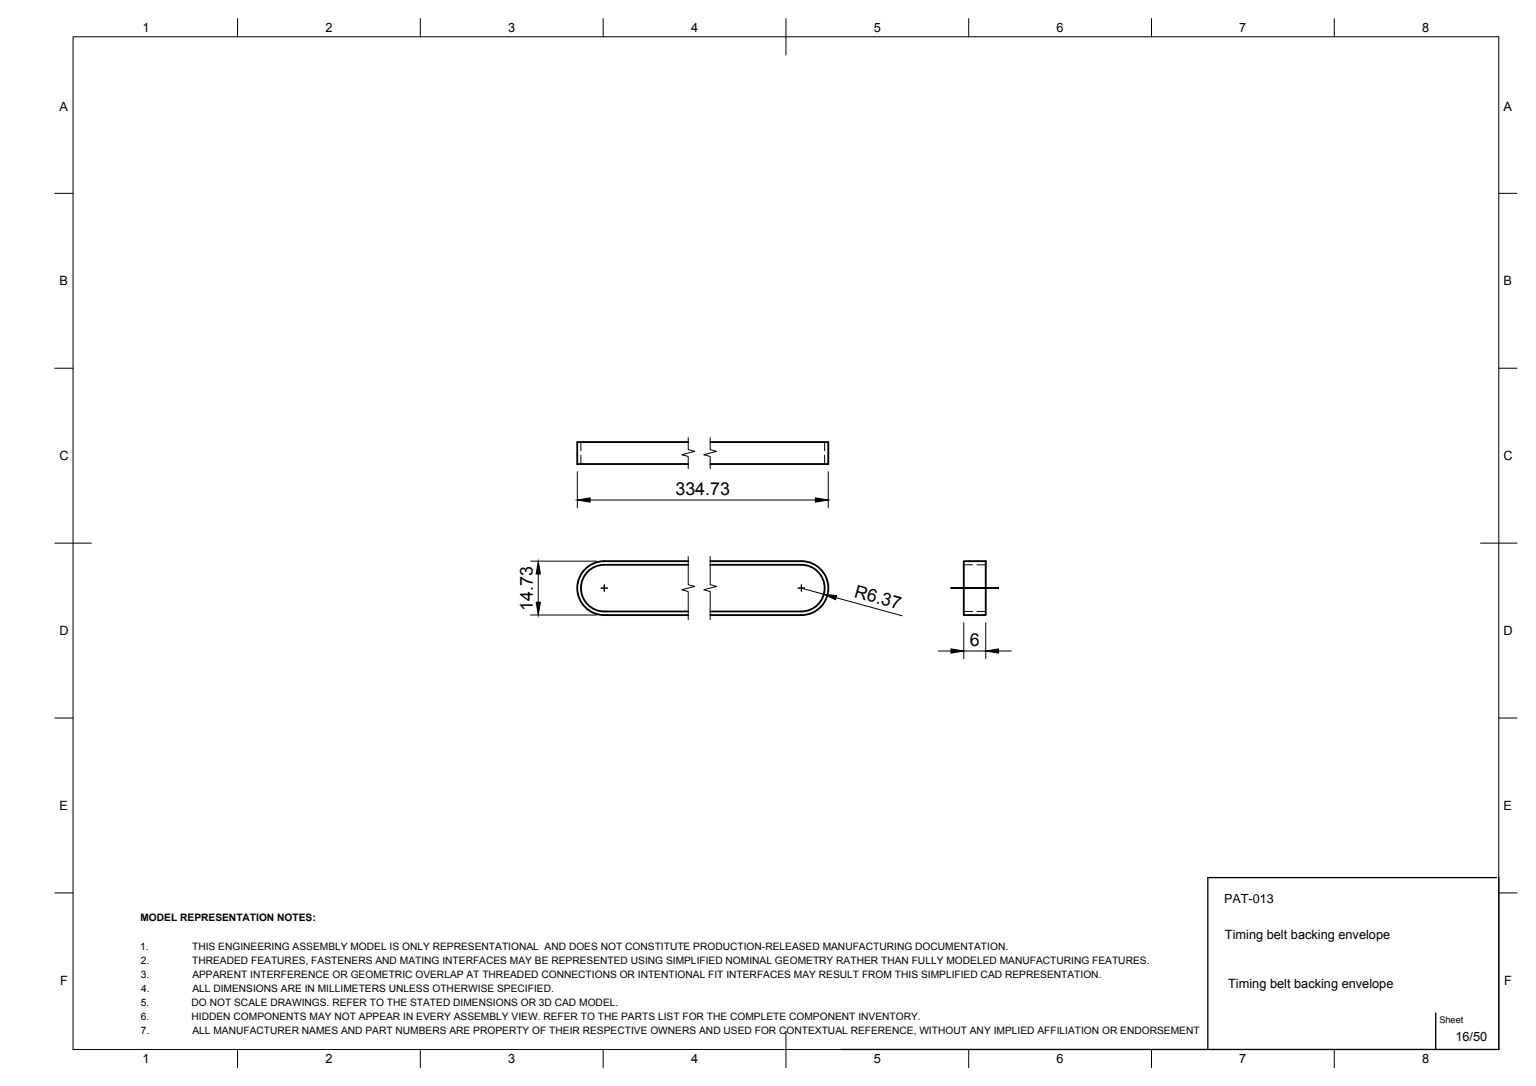
ISO-10303-21;
HEADER;
/* Generated by software containing ST-Developer
 * from STEP Tools, Inc. (www.steptools.com) 
 */

FILE_DESCRIPTION(
/* description */ ('Belt-driven linear axis on 2020 extrusion'),
/* implementation_level */ '2;1');

FILE_NAME(
/* name */ 'Timing belt backing envelope.step',
/* time_stamp */ '2026-10-28T03:26:09-07:00',
/* author */ (''),
/* organization */ (''),
/* preprocessor_version */ 'ST-DEVELOPER v20.2',
/* originating_system */ 'Autodesk Translation Framework v15.17.0.0',
/* authorisation */ '');

FILE_SCHEMA (('AUTOMOTIVE_DESIGN { 1 0 10303 214 3 1 1 }'));
ENDSEC;

DATA;
#10=MECHANICAL_DESIGN_GEOMETRIC_PRESENTATION_REPRESENTATION('',(#623),#20096);
#529=SHAPE_REPRESENTATION_RELATIONSHIP('SRR','None',#20325,#575);
#575=ADVANCED_BREP_SHAPE_REPRESENTATION('',(#679),#20056);
#623=STYLED_ITEM('',(#20657),#679);
#679=MANIFOLD_SOLID_BREP('Body1',#10936);
#794=FACE_BOUND('',#2115,.T.);
#795=FACE_BOUND('',#2123,.T.);
#971=PLANE('',#11832);
#972=PLANE('',#11833);
#973=PLANE('',#11834);
#974=PLANE('',#11845);
#975=PLANE('',#11846);
#976=PLANE('',#11849);
#1414=FACE_OUTER_BOUND('',#2112,.T.);
#1415=FACE_OUTER_BOUND('',#2113,.T.);
#1416=FACE_OUTER_BOUND('',#2114,.T.);
#1417=FACE_OUTER_BOUND('',#2116,.T.);
#1418=FACE_OUTER_BOUND('',#2117,.T.);
#1419=FACE_OUTER_BOUND('',#2118,.T.);
#1420=FACE_OUTER_BOUND('',#2119,.T.);
#1421=FACE_OUTER_BOUND('',#2120,.T.);
#1422=FACE_OUTER_BOUND('',#2121,.T.);
#1423=FACE_OUTER_BOUND('',#2122,.T.);
#2112=EDGE_LOOP('',(#7961,#7962,#7963,#7964));
#2113=EDGE_LOOP('',(#7965,#7966,#7967,#7968));
#2114=EDGE_LOOP('',(#7969,#7970,#7971,#7972));
#2115=EDGE_LOOP('',(#7973,#7974,#7975,#7976));
#2116=EDGE_LOOP('',(#7977,#7978,#7979,#7980));
#2117=EDGE_LOOP('',(#7981,#7982,#7983,#7984));
#2118=EDGE_LOOP('',(#7985,#7986,#7987,#7988));
#2119=EDGE_LOOP('',(#7989,#7990,#7991,#7992));
#2120=EDGE_LOOP('',(#7993,#7994,#7995,#7996));
#2121=EDGE_LOOP('',(#7997,#7998,#7999,#8000));
#2122=EDGE_LOOP('',(#8001,#8002,#8003,#8004));
#2123=EDGE_LOOP('',(#8005,#8006,#8007,#8008));
#2855=LINE('',#17003,#3712);
#2856=LINE('',#17005,#3713);
#2857=LINE('',#17007,#3714);
#2858=LINE('',#17008,#3715);
#2859=LINE('',#17012,#3716);
#2860=LINE('',#17014,#3717);
#2861=LINE('',#17016,#3718);
#2862=LINE('',#17017,#3719);
#2863=LINE('',#17021,#3720);
#2864=LINE('',#17025,#3721);
#2865=LINE('',#17035,#3722);
#2866=LINE('',#17038,#3723);
#2867=LINE('',#17041,#3724);
#2868=LINE('',#17042,#3725);
#2869=LINE('',#17045,#3726);
#2870=LINE('',#17046,#3727);
#3712=VECTOR('',#13661,1.);
#3713=VECTOR('',#13662,1.);
#3714=VECTOR('',#13663,1.);
#3715=VECTOR('',#13664,1.);
#3716=VECTOR('',#13667,1.);
#3717=VECTOR('',#13668,1.);
#3718=VECTOR('',#13669,1.);
#3719=VECTOR('',#13670,1.);
#3720=VECTOR('',#13673,1.);
#3721=VECTOR('',#13676,1.);
#3722=VECTOR('',#13693,1.);
#3723=VECTOR('',#13696,1.);
#3724=VECTOR('',#13699,1.);
#3725=VECTOR('',#13700,1.);
#3726=VECTOR('',#13703,1.);
#3727=VECTOR('',#13704,1.);
#4543=CIRCLE('',#11835,0.736619772367581);
#4544=CIRCLE('',#11836,0.736619772367582);
#4545=CIRCLE('',#11837,0.636619772367581);
#4546=CIRCLE('',#11838,0.636619772367581);
#4547=CIRCLE('',#11840,0.636619772367581);
#4548=CIRCLE('',#11842,0.636619772367581);
#4549=CIRCLE('',#11844,0.736619772367582);
#4550=CIRCLE('',#11848,0.736619772367581);
#5128=VERTEX_POINT('',#17001);
#5129=VERTEX_POINT('',#17002);
#5130=VERTEX_POINT('',#17004);
#5131=VERTEX_POINT('',#17006);
#5132=VERTEX_POINT('',#17010);
#5133=VERTEX_POINT('',#17011);
#5134=VERTEX_POINT('',#17013);
#5135=VERTEX_POINT('',#17015);
#5136=VERTEX_POINT('',#17019);
#5137=VERTEX_POINT('',#17020);
#5138=VERTEX_POINT('',#17022);
#5139=VERTEX_POINT('',#17024);
#5140=VERTEX_POINT('',#17034);
#5141=VERTEX_POINT('',#17036);
#5142=VERTEX_POINT('',#17040);
#5143=VERTEX_POINT('',#17044);
#6195=EDGE_CURVE('',#5128,#5129,#2855,.T.);
#6196=EDGE_CURVE('',#5130,#5128,#2856,.T.);
#6197=EDGE_CURVE('',#5131,#5130,#2857,.T.);
#6198=EDGE_CURVE('',#5131,#5129,#2858,.T.);
#6199=EDGE_CURVE('',#5132,#5133,#2859,.T.);
#6200=EDGE_CURVE('',#5134,#5132,#2860,.T.);
#6201=EDGE_CURVE('',#5135,#5134,#2861,.T.);
#6202=EDGE_CURVE('',#5133,#5135,#2862,.T.);
#6203=EDGE_CURVE('',#5136,#5137,#2863,.T.);
#6204=EDGE_CURVE('',#5138,#5136,#4543,.T.);
#6205=EDGE_CURVE('',#5139,#5138,#2864,.T.);
#6206=EDGE_CURVE('',#5137,#5139,#4544,.T.);
#6207=EDGE_CURVE('',#5129,#5132,#4545,.T.);
#6208=EDGE_CURVE('',#5133,#5128,#4546,.T.);
#6209=EDGE_CURVE('',#5134,#5131,#4547,.T.);
#6210=EDGE_CURVE('',#5130,#5135,#4548,.T.);
#6211=EDGE_CURVE('',#5139,#5140,#2865,.T.);
#6212=EDGE_CURVE('',#5141,#5140,#4549,.T.);
#6213=EDGE_CURVE('',#5137,#5141,#2866,.T.);
#6214=EDGE_CURVE('',#5138,#5142,#2867,.T.);
#6215=EDGE_CURVE('',#5140,#5142,#2868,.T.);
#6216=EDGE_CURVE('',#5143,#5141,#2869,.T.);
#6217=EDGE_CURVE('',#5136,#5143,#2870,.T.);
#6218=EDGE_CURVE('',#5142,#5143,#4550,.T.);
#7961=ORIENTED_EDGE('',*,*,#6195,.F.);
#7962=ORIENTED_EDGE('',*,*,#6196,.F.);
#7963=ORIENTED_EDGE('',*,*,#6197,.F.);
#7964=ORIENTED_EDGE('',*,*,#6198,.T.);
#7965=ORIENTED_EDGE('',*,*,#6199,.F.);
#7966=ORIENTED_EDGE('',*,*,#6200,.F.);
#7967=ORIENTED_EDGE('',*,*,#6201,.F.);
#7968=ORIENTED_EDGE('',*,*,#6202,.F.);
#7969=ORIENTED_EDGE('',*,*,#6203,.F.);
#7970=ORIENTED_EDGE('',*,*,#6204,.F.);
#7971=ORIENTED_EDGE('',*,*,#6205,.F.);
#7972=ORIENTED_EDGE('',*,*,#6206,.F.);
#7973=ORIENTED_EDGE('',*,*,#6195,.T.);
#7974=ORIENTED_EDGE('',*,*,#6207,.T.);
#7975=ORIENTED_EDGE('',*,*,#6199,.T.);
#7976=ORIENTED_EDGE('',*,*,#6208,.T.);
#7977=ORIENTED_EDGE('',*,*,#6198,.F.);
#7978=ORIENTED_EDGE('',*,*,#6209,.F.);
#7979=ORIENTED_EDGE('',*,*,#6200,.T.);
#7980=ORIENTED_EDGE('',*,*,#6207,.F.);
#7981=ORIENTED_EDGE('',*,*,#6196,.T.);
#7982=ORIENTED_EDGE('',*,*,#6208,.F.);
#7983=ORIENTED_EDGE('',*,*,#6202,.T.);
#7984=ORIENTED_EDGE('',*,*,#6210,.F.);
#7985=ORIENTED_EDGE('',*,*,#6211,.T.);
#7986=ORIENTED_EDGE('',*,*,#6212,.F.);
#7987=ORIENTED_EDGE('',*,*,#6213,.F.);
#7988=ORIENTED_EDGE('',*,*,#6206,.T.);
#7989=ORIENTED_EDGE('',*,*,#6205,.T.);
#7990=ORIENTED_EDGE('',*,*,#6214,.T.);
#7991=ORIENTED_EDGE('',*,*,#6215,.F.);
#7992=ORIENTED_EDGE('',*,*,#6211,.F.);
#7993=ORIENTED_EDGE('',*,*,#6203,.T.);
#7994=ORIENTED_EDGE('',*,*,#6213,.T.);
#7995=ORIENTED_EDGE('',*,*,#6216,.F.);
#7996=ORIENTED_EDGE('',*,*,#6217,.F.);
#7997=ORIENTED_EDGE('',*,*,#6214,.F.);
#7998=ORIENTED_EDGE('',*,*,#6204,.T.);
#7999=ORIENTED_EDGE('',*,*,#6217,.T.);
#8000=ORIENTED_EDGE('',*,*,#6218,.F.);
#8001=ORIENTED_EDGE('',*,*,#6215,.T.);
#8002=ORIENTED_EDGE('',*,*,#6218,.T.);
#8003=ORIENTED_EDGE('',*,*,#6216,.T.);
#8004=ORIENTED_EDGE('',*,*,#6212,.T.);
#8005=ORIENTED_EDGE('',*,*,#6197,.T.);
#8006=ORIENTED_EDGE('',*,*,#6210,.T.);
#8007=ORIENTED_EDGE('',*,*,#6201,.T.);
#8008=ORIENTED_EDGE('',*,*,#6209,.T.);
#10159=CYLINDRICAL_SURFACE('',#11839,0.636619772367581);
#10160=CYLINDRICAL_SURFACE('',#11841,0.636619772367581);
#10161=CYLINDRICAL_SURFACE('',#11843,0.736619772367582);
#10162=CYLINDRICAL_SURFACE('',#11847,0.736619772367581);
#10465=ADVANCED_FACE('',(#1414),#971,.F.);
#10466=ADVANCED_FACE('',(#1415),#972,.F.);
#10467=ADVANCED_FACE('',(#1416,#794),#973,.F.);
#10468=ADVANCED_FACE('',(#1417),#10159,.F.);
#10469=ADVANCED_FACE('',(#1418),#10160,.F.);
#10470=ADVANCED_FACE('',(#1419),#10161,.T.);
#10471=ADVANCED_FACE('',(#1420),#974,.T.);
#10472=ADVANCED_FACE('',(#1421),#975,.T.);
#10473=ADVANCED_FACE('',(#1422),#10162,.T.);
#10474=ADVANCED_FACE('',(#1423,#795),#976,.T.);
#10936=CLOSED_SHELL('',(#10465,#10466,#10467,#10468,#10469,#10470,#10471,
#10472,#10473,#10474));
#11831=AXIS2_PLACEMENT_3D('',#16999,#13657,#13658);
#11832=AXIS2_PLACEMENT_3D('',#17000,#13659,#13660);
#11833=AXIS2_PLACEMENT_3D('',#17009,#13665,#13666);
#11834=AXIS2_PLACEMENT_3D('',#17018,#13671,#13672);
#11835=AXIS2_PLACEMENT_3D('',#17023,#13674,#13675);
#11836=AXIS2_PLACEMENT_3D('',#17026,#13677,#13678);
#11837=AXIS2_PLACEMENT_3D('',#17027,#13679,#13680);
#11838=AXIS2_PLACEMENT_3D('',#17028,#13681,#13682);
#11839=AXIS2_PLACEMENT_3D('',#17029,#13683,#13684);
#11840=AXIS2_PLACEMENT_3D('',#17030,#13685,#13686);
#11841=AXIS2_PLACEMENT_3D('',#17031,#13687,#13688);
#11842=AXIS2_PLACEMENT_3D('',#17032,#13689,#13690);
#11843=AXIS2_PLACEMENT_3D('',#17033,#13691,#13692);
#11844=AXIS2_PLACEMENT_3D('',#17037,#13694,#13695);
#11845=AXIS2_PLACEMENT_3D('',#17039,#13697,#13698);
#11846=AXIS2_PLACEMENT_3D('',#17043,#13701,#13702);
#11847=AXIS2_PLACEMENT_3D('',#17047,#13705,#13706);
#11848=AXIS2_PLACEMENT_3D('',#17048,#13707,#13708);
#11849=AXIS2_PLACEMENT_3D('',#17049,#13709,#13710);
#13657=DIRECTION('axis',(0.,0.,1.));
#13658=DIRECTION('refdir',(1.,0.,0.));
#13659=DIRECTION('center_axis',(0.,0.,-1.));
#13660=DIRECTION('ref_axis',(-1.,0.,0.));
#13661=DIRECTION('',(-1.,0.,0.));
#13662=DIRECTION('',(0.,-1.,0.));
#13663=DIRECTION('',(1.,0.,0.));
#13664=DIRECTION('',(0.,-1.,0.));
#13665=DIRECTION('center_axis',(0.,0.,1.));
#13666=DIRECTION('ref_axis',(1.,0.,0.));
#13667=DIRECTION('',(1.,0.,0.));
#13668=DIRECTION('',(0.,-1.,0.));
#13669=DIRECTION('',(-1.,0.,0.));
#13670=DIRECTION('',(0.,1.,0.));
#13671=DIRECTION('center_axis',(0.,1.,0.));
#13672=DIRECTION('ref_axis',(1.,0.,0.));
#13673=DIRECTION('',(1.,0.,0.));
#13674=DIRECTION('center_axis',(0.,1.,0.));
#13675=DIRECTION('ref_axis',(1.,0.,0.));
#13676=DIRECTION('',(-1.,0.,0.));
#13677=DIRECTION('center_axis',(0.,1.,0.));
#13678=DIRECTION('ref_axis',(1.,0.,0.));
#13679=DIRECTION('center_axis',(0.,1.,0.));
#13680=DIRECTION('ref_axis',(1.,0.,0.));
#13681=DIRECTION('center_axis',(0.,1.,0.));
#13682=DIRECTION('ref_axis',(1.,0.,0.));
#13683=DIRECTION('center_axis',(0.,1.,0.));
#13684=DIRECTION('ref_axis',(-1.,0.,-1.22464679914735E-16));
#13685=DIRECTION('center_axis',(0.,-1.,0.));
#13686=DIRECTION('ref_axis',(1.,0.,0.));
#13687=DIRECTION('center_axis',(0.,1.,0.));
#13688=DIRECTION('ref_axis',(1.,0.,0.));
#13689=DIRECTION('center_axis',(0.,-1.,0.));
#13690=DIRECTION('ref_axis',(1.,0.,0.));
#13691=DIRECTION('center_axis',(0.,1.,0.));
#13692=DIRECTION('ref_axis',(1.,0.,0.));
#13693=DIRECTION('',(0.,1.,0.));
#13694=DIRECTION('center_axis',(0.,1.,0.));
#13695=DIRECTION('ref_axis',(1.,0.,0.));
#13696=DIRECTION('',(0.,1.,0.));
#13697=DIRECTION('center_axis',(0.,0.,-1.));
#13698=DIRECTION('ref_axis',(-1.,0.,0.));
#13699=DIRECTION('',(0.,1.,0.));
#13700=DIRECTION('',(-1.,0.,0.));
#13701=DIRECTION('center_axis',(0.,0.,1.));
#13702=DIRECTION('ref_axis',(1.,0.,0.));
#13703=DIRECTION('',(1.,0.,0.));
#13704=DIRECTION('',(0.,1.,0.));
#13705=DIRECTION('center_axis',(0.,1.,0.));
#13706=DIRECTION('ref_axis',(-1.,0.,-1.22464679914735E-16));
#13707=DIRECTION('center_axis',(0.,1.,0.));
#13708=DIRECTION('ref_axis',(1.,0.,0.));
#13709=DIRECTION('center_axis',(0.,1.,0.));
#13710=DIRECTION('ref_axis',(1.,0.,0.));
#16999=CARTESIAN_POINT('',(0.,0.,0.));
#17000=CARTESIAN_POINT('Origin',(32.,-3.5,6.36338022763242));
#17001=CARTESIAN_POINT('',(32.,-3.425,6.36338022763242));
#17002=CARTESIAN_POINT('',(0.,-3.425,6.36338022763242));
#17003=CARTESIAN_POINT('',(16.,-3.425,6.36338022763242));
#17004=CARTESIAN_POINT('',(32.,-2.825,6.36338022763242));
#17005=CARTESIAN_POINT('',(32.,-3.5,6.36338022763242));
#17006=CARTESIAN_POINT('',(0.,-2.825,6.36338022763242));
#17007=CARTESIAN_POINT('',(16.,-2.825,6.36338022763242));
#17008=CARTESIAN_POINT('',(0.,-3.5,6.36338022763242));
#17009=CARTESIAN_POINT('Origin',(0.,-3.5,7.63661977236758));
#17010=CARTESIAN_POINT('',(0.,-3.425,7.63661977236758));
#17011=CARTESIAN_POINT('',(32.,-3.425,7.63661977236758));
#17012=CARTESIAN_POINT('',(0.,-3.425,7.63661977236758));
#17013=CARTESIAN_POINT('',(0.,-2.825,7.63661977236758));
#17014=CARTESIAN_POINT('',(0.,-3.5,7.63661977236758));
#17015=CARTESIAN_POINT('',(32.,-2.825,7.63661977236758));
#17016=CARTESIAN_POINT('',(0.,-2.825,7.63661977236758));
#17017=CARTESIAN_POINT('',(32.,-3.5,7.63661977236758));
#17018=CARTESIAN_POINT('Origin',(0.,-3.425,7.));
#17019=CARTESIAN_POINT('',(0.,-3.425,7.73661977236758));
#17020=CARTESIAN_POINT('',(32.,-3.425,7.73661977236758));
#17021=CARTESIAN_POINT('',(0.,-3.425,7.73661977236758));
#17022=CARTESIAN_POINT('',(0.,-3.425,6.26338022763242));
#17023=CARTESIAN_POINT('Origin',(0.,-3.425,7.));
#17024=CARTESIAN_POINT('',(32.,-3.425,6.26338022763242));
#17025=CARTESIAN_POINT('',(32.,-3.425,6.26338022763242));
#17026=CARTESIAN_POINT('Origin',(32.,-3.425,7.));
#17027=CARTESIAN_POINT('Origin',(0.,-3.425,7.));
#17028=CARTESIAN_POINT('Origin',(32.,-3.425,7.));
#17029=CARTESIAN_POINT('Origin',(0.,-3.5,7.));
#17030=CARTESIAN_POINT('Origin',(0.,-2.825,7.));
#17031=CARTESIAN_POINT('Origin',(32.,-3.5,7.));
#17032=CARTESIAN_POINT('Origin',(32.,-2.825,7.));
#17033=CARTESIAN_POINT('Origin',(32.,-3.425,7.));
#17034=CARTESIAN_POINT('',(32.,-2.825,6.26338022763242));
#17035=CARTESIAN_POINT('',(32.,-3.425,6.26338022763242));
#17036=CARTESIAN_POINT('',(32.,-2.825,7.73661977236758));
#17037=CARTESIAN_POINT('Origin',(32.,-2.825,7.));
#17038=CARTESIAN_POINT('',(32.,-3.425,7.73661977236758));
#17039=CARTESIAN_POINT('Origin',(32.,-3.425,6.26338022763242));
#17040=CARTESIAN_POINT('',(0.,-2.825,6.26338022763242));
#17041=CARTESIAN_POINT('',(0.,-3.425,6.26338022763242));
#17042=CARTESIAN_POINT('',(32.,-2.825,6.26338022763242));
#17043=CARTESIAN_POINT('Origin',(0.,-3.425,7.73661977236758));
#17044=CARTESIAN_POINT('',(0.,-2.825,7.73661977236758));
#17045=CARTESIAN_POINT('',(0.,-2.825,7.73661977236758));
#17046=CARTESIAN_POINT('',(0.,-3.425,7.73661977236758));
#17047=CARTESIAN_POINT('Origin',(0.,-3.425,7.));
#17048=CARTESIAN_POINT('Origin',(0.,-2.825,7.));
#17049=CARTESIAN_POINT('Origin',(0.,-2.825,7.));
#20002=UNCERTAINTY_MEASURE_WITH_UNIT(LENGTH_MEASURE(0.001),#20097,
'DISTANCE_ACCURACY_VALUE',
'Maximum model space distance between geometric entities at asserted c
onnectivities');
#20042=UNCERTAINTY_MEASURE_WITH_UNIT(LENGTH_MEASURE(0.001),#20097,
'DISTANCE_ACCURACY_VALUE',
'Maximum model space distance between geometric entities at asserted c
onnectivities');
#20056=(
GEOMETRIC_REPRESENTATION_CONTEXT(3)
GLOBAL_UNCERTAINTY_ASSIGNED_CONTEXT((#20002))
GLOBAL_UNIT_ASSIGNED_CONTEXT((#20097,#20099,#20100))
REPRESENTATION_CONTEXT('','3D')
);
#20096=(
GEOMETRIC_REPRESENTATION_CONTEXT(3)
GLOBAL_UNCERTAINTY_ASSIGNED_CONTEXT((#20042))
GLOBAL_UNIT_ASSIGNED_CONTEXT((#20097,#20099,#20100))
REPRESENTATION_CONTEXT('','3D')
);
#20097=(
LENGTH_UNIT()
NAMED_UNIT(*)
SI_UNIT(.CENTI.,.METRE.)
);
#20099=(
NAMED_UNIT(*)
PLANE_ANGLE_UNIT()
SI_UNIT($,.RADIAN.)
);
#20100=(
NAMED_UNIT(*)
SI_UNIT($,.STERADIAN.)
SOLID_ANGLE_UNIT()
);
#20114=SHAPE_DEFINITION_REPRESENTATION(#20167,#20325);
#20167=PRODUCT_DEFINITION_SHAPE('',$,#20379);
#20325=SHAPE_REPRESENTATION('',(#11831),#20056);
#20365=PRODUCT_DEFINITION_CONTEXT('part definition',#20526,'design');
#20379=PRODUCT_DEFINITION('Timing belt backing envelope',
'Timing belt backing envelope',#20432,#20365);
#20432=PRODUCT_DEFINITION_FORMATION('',$,#20541);
#20526=APPLICATION_CONTEXT(
'Core Data for Automotive Mechanical Design Process');
#20527=PRODUCT_CONTEXT('part definition',#20526,'mechanical');
#20541=PRODUCT('Timing belt backing envelope',
'Timing belt backing envelope','Timing belt backing envelope',(#20527));
#20651=COLOUR_RGB('Black',0.12,0.14,0.17);
#20652=FILL_AREA_STYLE_COLOUR('',#20651);
#20653=FILL_AREA_STYLE('',(#20652));
#20654=SURFACE_STYLE_FILL_AREA(#20653);
#20655=SURFACE_SIDE_STYLE('',(#20654));
#20656=SURFACE_STYLE_USAGE(.BOTH.,#20655);
#20657=PRESENTATION_STYLE_ASSIGNMENT((#20656));
ENDSEC;
END-ISO-10303-21;
